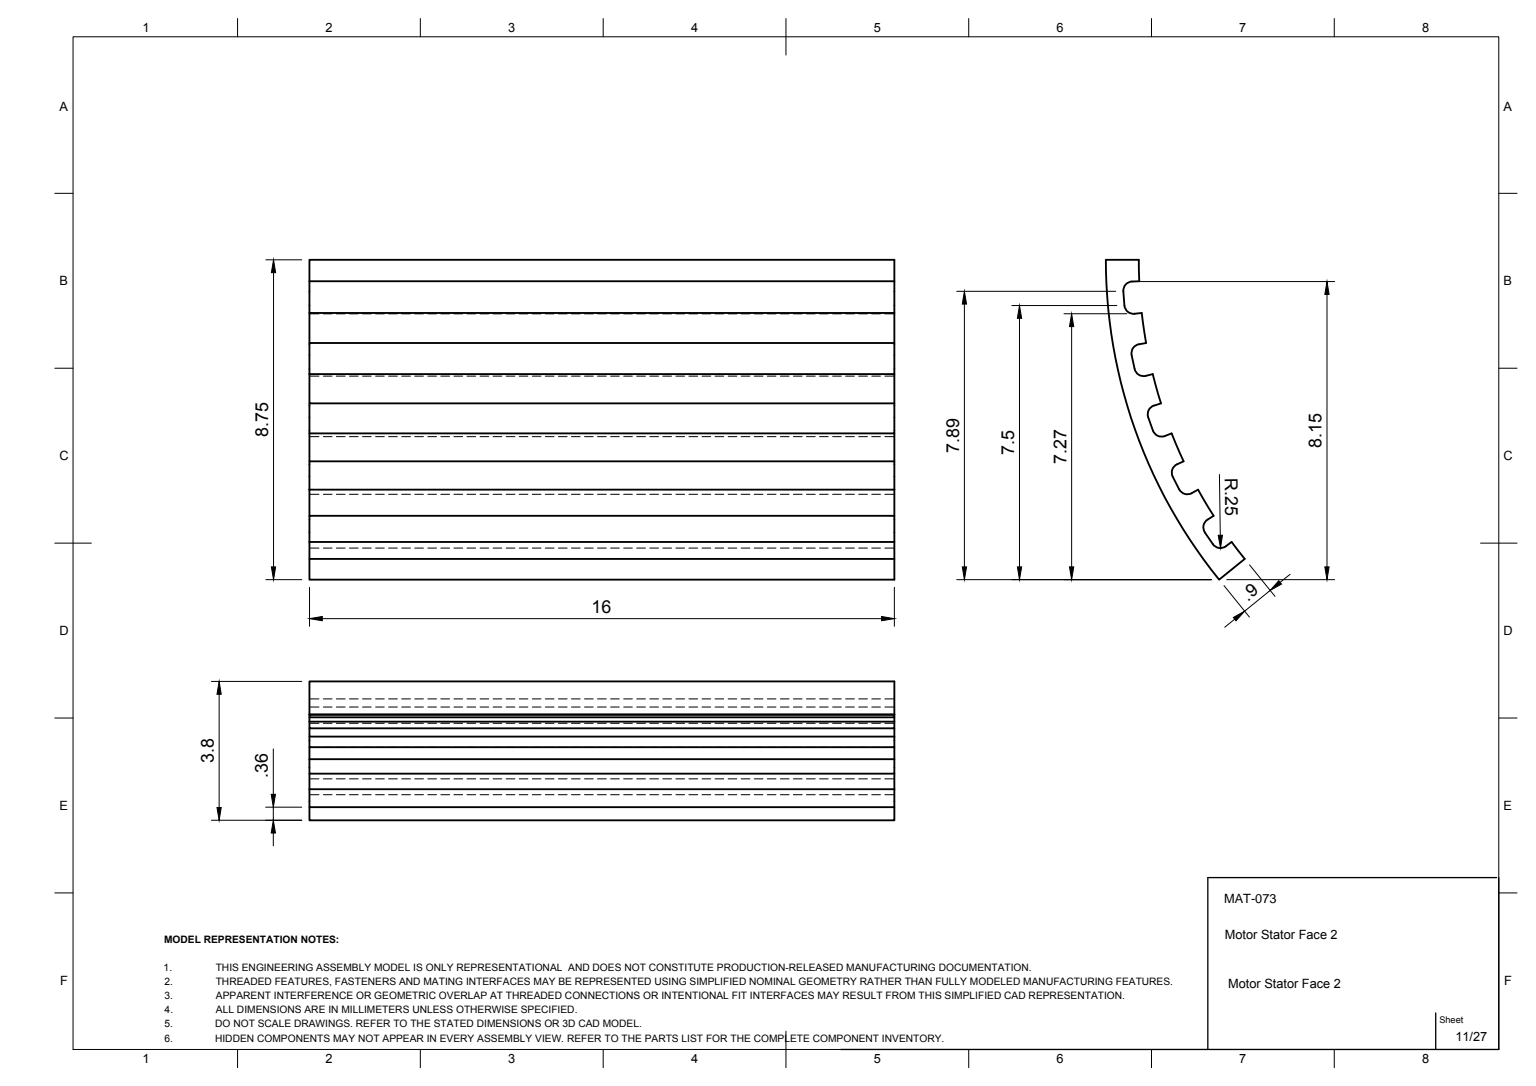
ISO-10303-21;
HEADER;
/* Generated by software containing ST-Developer
 * from STEP Tools, Inc. (www.steptools.com) 
 */

FILE_DESCRIPTION(
/* description */ ('CAx-IF Rec.Pracs.---Representation and Presentation of Product Manufa
cturing Information (PMI)---4.0---2014-10-13'),
/* implementation_level */ '2;1');

FILE_NAME(
/* name */ 'Motor Stator Face 2.step',
/* time_stamp */ '2026-10-24T18:52:33-07:00',
/* author */ (''),
/* organization */ (''),
/* preprocessor_version */ 'ST-DEVELOPER v20.2',
/* originating_system */ 'Autodesk Translation Framework v15.17.0.0',
/* authorisation */ '');

FILE_SCHEMA (('AP242_MANAGED_MODEL_BASED_3D_ENGINEERING_MIM_LF { 1 0 10303 442 2 1 4 }'));
ENDSEC;

DATA;
#10=MECHANICAL_DESIGN_GEOMETRIC_PRESENTATION_REPRESENTATION('',(#424),#34876);
#358=SHAPE_REPRESENTATION_RELATIONSHIP('SRR','None',#34995,#391);
#391=ADVANCED_BREP_SHAPE_REPRESENTATION('',(#457),#34853);
#424=STYLED_ITEM('',(#35166),#457);
#457=MANIFOLD_SOLID_BREP('Motor Stator Face 2',#19564);
#802=PLANE('',#20894);
#803=PLANE('',#20904);
#804=PLANE('',#20914);
#805=PLANE('',#20924);
#806=PLANE('',#20934);
#807=PLANE('',#20935);
#808=PLANE('',#20936);
#809=PLANE('',#20937);
#810=PLANE('',#20938);
#811=PLANE('',#20945);
#812=PLANE('',#20955);
#813=PLANE('',#20958);
#814=PLANE('',#20961);
#815=PLANE('',#20964);
#1709=LINE('',#31107,#3308);
#1710=LINE('',#31110,#3309);
#1711=LINE('',#31115,#3310);
#1712=LINE('',#31121,#3311);
#1713=LINE('',#31125,#3312);
#1714=LINE('',#31127,#3313);
#1715=LINE('',#31128,#3314);
#1716=LINE('',#31134,#3315);
#1717=LINE('',#31137,#3316);
#1718=LINE('',#31142,#3317);
#1719=LINE('',#31148,#3318);
#1720=LINE('',#31152,#3319);
#1721=LINE('',#31154,#3320);
#1722=LINE('',#31155,#3321);
#1723=LINE('',#31161,#3322);
#1724=LINE('',#31164,#3323);
#1725=LINE('',#31169,#3324);
#1726=LINE('',#31175,#3325);
#1727=LINE('',#31179,#3326);
#1728=LINE('',#31181,#3327);
#1729=LINE('',#31182,#3328);
#1730=LINE('',#31188,#3329);
#1731=LINE('',#31191,#3330);
#1732=LINE('',#31196,#3331);
#1733=LINE('',#31202,#3332);
#1734=LINE('',#31206,#3333);
#1735=LINE('',#31208,#3334);
#1736=LINE('',#31209,#3335);
#1737=LINE('',#31215,#3336);
#1738=LINE('',#31218,#3337);
#1739=LINE('',#31223,#3338);
#1740=LINE('',#31229,#3339);
#1741=LINE('',#31233,#3340);
#1742=LINE('',#31235,#3341);
#1743=LINE('',#31236,#3342);
#1744=LINE('',#31239,#3343);
#1745=LINE('',#31241,#3344);
#1746=LINE('',#31242,#3345);
#1747=LINE('',#31245,#3346);
#1748=LINE('',#31247,#3347);
#1749=LINE('',#31248,#3348);
#1750=LINE('',#31251,#3349);
#1751=LINE('',#31253,#3350);
#1752=LINE('',#31254,#3351);
#1753=LINE('',#31257,#3352);
#1754=LINE('',#31259,#3353);
#1755=LINE('',#31260,#3354);
#1756=LINE('',#31265,#3355);
#1757=LINE('',#31272,#3356);
#1758=LINE('',#31276,#3357);
#1759=LINE('',#31281,#3358);
#1760=LINE('',#31286,#3359);
#1761=LINE('',#31289,#3360);
#1762=LINE('',#31292,#3361);
#1763=LINE('',#31297,#3362);
#1764=LINE('',#31298,#3363);
#1765=LINE('',#31302,#3364);
#1766=LINE('',#31304,#3365);
#3308=VECTOR('',#24756,1.);
#3309=VECTOR('',#24759,1.);
#3310=VECTOR('',#24764,1.);
#3311=VECTOR('',#24771,1.);
#3312=VECTOR('',#24776,1.);
#3313=VECTOR('',#24777,1.);
#3314=VECTOR('',#24778,1.);
#3315=VECTOR('',#24783,1.);
#3316=VECTOR('',#24786,1.);
#3317=VECTOR('',#24791,1.);
#3318=VECTOR('',#24798,1.);
#3319=VECTOR('',#24803,1.);
#3320=VECTOR('',#24804,1.);
#3321=VECTOR('',#24805,1.);
#3322=VECTOR('',#24810,1.);
#3323=VECTOR('',#24813,1.);
#3324=VECTOR('',#24818,1.);
#3325=VECTOR('',#24825,1.);
#3326=VECTOR('',#24830,1.);
#3327=VECTOR('',#24831,1.);
#3328=VECTOR('',#24832,1.);
#3329=VECTOR('',#24837,1.);
#3330=VECTOR('',#24840,1.);
#3331=VECTOR('',#24845,1.);
#3332=VECTOR('',#24852,1.);
#3333=VECTOR('',#24857,1.);
#3334=VECTOR('',#24858,1.);
#3335=VECTOR('',#24859,1.);
#3336=VECTOR('',#24864,1.);
#3337=VECTOR('',#24867,1.);
#3338=VECTOR('',#24872,1.);
#3339=VECTOR('',#24879,1.);
#3340=VECTOR('',#24884,1.);
#3341=VECTOR('',#24885,1.);
#3342=VECTOR('',#24886,1.);
#3343=VECTOR('',#24889,1.);
#3344=VECTOR('',#24890,1.);
#3345=VECTOR('',#24891,1.);
#3346=VECTOR('',#24894,1.);
#3347=VECTOR('',#24895,1.);
#3348=VECTOR('',#24896,1.);
#3349=VECTOR('',#24899,1.);
#3350=VECTOR('',#24900,1.);
#3351=VECTOR('',#24901,1.);
#3352=VECTOR('',#24904,1.);
#3353=VECTOR('',#24905,1.);
#3354=VECTOR('',#24906,1.);
#3355=VECTOR('',#24911,1.);
#3356=VECTOR('',#24922,1.);
#3357=VECTOR('',#24925,1.);
#3358=VECTOR('',#24932,1.);
#3359=VECTOR('',#24939,1.);
#3360=VECTOR('',#24942,1.);
#3361=VECTOR('',#24947,1.);
#3362=VECTOR('',#24954,1.);
#3363=VECTOR('',#24955,1.);
#3364=VECTOR('',#24960,1.);
#3365=VECTOR('',#24963,1.);
#4482=CYLINDRICAL_SURFACE('',#20885,0.00025);
#4483=CYLINDRICAL_SURFACE('',#20888,0.01345);
#4484=CYLINDRICAL_SURFACE('',#20891,0.00025);
#4485=CYLINDRICAL_SURFACE('',#20895,0.00025);
#4486=CYLINDRICAL_SURFACE('',#20898,0.01345);
#4487=CYLINDRICAL_SURFACE('',#20901,0.00025);
#4488=CYLINDRICAL_SURFACE('',#20905,0.00025);
#4489=CYLINDRICAL_SURFACE('',#20908,0.01345);
#4490=CYLINDRICAL_SURFACE('',#20911,0.00025);
#4491=CYLINDRICAL_SURFACE('',#20915,0.00025);
#4492=CYLINDRICAL_SURFACE('',#20918,0.01345);
#4493=CYLINDRICAL_SURFACE('',#20921,0.00025);
#4494=CYLINDRICAL_SURFACE('',#20925,0.00025);
#4495=CYLINDRICAL_SURFACE('',#20928,0.01345);
#4496=CYLINDRICAL_SURFACE('',#20931,0.00025);
#4497=CYLINDRICAL_SURFACE('',#20939,0.013);
#4498=CYLINDRICAL_SURFACE('',#20942,0.013);
#4499=CYLINDRICAL_SURFACE('',#20951,0.013);
#4500=CYLINDRICAL_SURFACE('',#20953,0.013);
#4501=CYLINDRICAL_SURFACE('',#20956,0.013);
#4502=CYLINDRICAL_SURFACE('',#20959,0.0139);
#4503=CYLINDRICAL_SURFACE('',#20962,0.013);
#5216=FACE_OUTER_BOUND('',#6300,.T.);
#5217=FACE_OUTER_BOUND('',#6301,.T.);
#5218=FACE_OUTER_BOUND('',#6302,.T.);
#5219=FACE_OUTER_BOUND('',#6303,.T.);
#5220=FACE_OUTER_BOUND('',#6304,.T.);
#5221=FACE_OUTER_BOUND('',#6305,.T.);
#5222=FACE_OUTER_BOUND('',#6306,.T.);
#5223=FACE_OUTER_BOUND('',#6307,.T.);
#5224=FACE_OUTER_BOUND('',#6308,.T.);
#5225=FACE_OUTER_BOUND('',#6309,.T.);
#5226=FACE_OUTER_BOUND('',#6310,.T.);
#5227=FACE_OUTER_BOUND('',#6311,.T.);
#5228=FACE_OUTER_BOUND('',#6312,.T.);
#5229=FACE_OUTER_BOUND('',#6313,.T.);
#5230=FACE_OUTER_BOUND('',#6314,.T.);
#5231=FACE_OUTER_BOUND('',#6315,.T.);
#5232=FACE_OUTER_BOUND('',#6316,.T.);
#5233=FACE_OUTER_BOUND('',#6317,.T.);
#5234=FACE_OUTER_BOUND('',#6318,.T.);
#5235=FACE_OUTER_BOUND('',#6319,.T.);
#5236=FACE_OUTER_BOUND('',#6320,.T.);
#5237=FACE_OUTER_BOUND('',#6321,.T.);
#5238=FACE_OUTER_BOUND('',#6322,.T.);
#5239=FACE_OUTER_BOUND('',#6323,.T.);
#5240=FACE_OUTER_BOUND('',#6324,.T.);
#5241=FACE_OUTER_BOUND('',#6325,.T.);
#5242=FACE_OUTER_BOUND('',#6326,.T.);
#5243=FACE_OUTER_BOUND('',#6327,.T.);
#5244=FACE_OUTER_BOUND('',#6328,.T.);
#5245=FACE_OUTER_BOUND('',#6329,.T.);
#5246=FACE_OUTER_BOUND('',#6330,.T.);
#5247=FACE_OUTER_BOUND('',#6331,.T.);
#5248=FACE_OUTER_BOUND('',#6332,.T.);
#5249=FACE_OUTER_BOUND('',#6333,.T.);
#5250=FACE_OUTER_BOUND('',#6334,.T.);
#5251=FACE_OUTER_BOUND('',#6335,.T.);
#6300=EDGE_LOOP('',(#15096,#15097,#15098,#15099));
#6301=EDGE_LOOP('',(#15100,#15101,#15102,#15103));
#6302=EDGE_LOOP('',(#15104,#15105,#15106,#15107));
#6303=EDGE_LOOP('',(#15108,#15109,#15110,#15111));
#6304=EDGE_LOOP('',(#15112,#15113,#15114,#15115));
#6305=EDGE_LOOP('',(#15116,#15117,#15118,#15119));
#6306=EDGE_LOOP('',(#15120,#15121,#15122,#15123));
#6307=EDGE_LOOP('',(#15124,#15125,#15126,#15127));
#6308=EDGE_LOOP('',(#15128,#15129,#15130,#15131));
#6309=EDGE_LOOP('',(#15132,#15133,#15134,#15135));
#6310=EDGE_LOOP('',(#15136,#15137,#15138,#15139));
#6311=EDGE_LOOP('',(#15140,#15141,#15142,#15143));
#6312=EDGE_LOOP('',(#15144,#15145,#15146,#15147));
#6313=EDGE_LOOP('',(#15148,#15149,#15150,#15151));
#6314=EDGE_LOOP('',(#15152,#15153,#15154,#15155));
#6315=EDGE_LOOP('',(#15156,#15157,#15158,#15159));
#6316=EDGE_LOOP('',(#15160,#15161,#15162,#15163));
#6317=EDGE_LOOP('',(#15164,#15165,#15166,#15167));
#6318=EDGE_LOOP('',(#15168,#15169,#15170,#15171));
#6319=EDGE_LOOP('',(#15172,#15173,#15174,#15175));
#6320=EDGE_LOOP('',(#15176,#15177,#15178,#15179));
#6321=EDGE_LOOP('',(#15180,#15181,#15182,#15183));
#6322=EDGE_LOOP('',(#15184,#15185,#15186,#15187));
#6323=EDGE_LOOP('',(#15188,#15189,#15190,#15191));
#6324=EDGE_LOOP('',(#15192,#15193,#15194,#15195));
#6325=EDGE_LOOP('',(#15196,#15197,#15198,#15199));
#6326=EDGE_LOOP('',(#15200,#15201,#15202,#15203,#15204,#15205,#15206,#15207,
#15208,#15209,#15210,#15211,#15212,#15213,#15214,#15215,#15216,#15217,#15218,
#15219,#15220,#15221,#15222,#15223,#15224,#15225,#15226,#15227,#15228,#15229,
#15230,#15231,#15232,#15233));
#6327=EDGE_LOOP('',(#15234,#15235,#15236,#15237));
#6328=EDGE_LOOP('',(#15238,#15239,#15240,#15241));
#6329=EDGE_LOOP('',(#15242,#15243,#15244,#15245));
#6330=EDGE_LOOP('',(#15246,#15247,#15248,#15249));
#6331=EDGE_LOOP('',(#15250,#15251,#15252,#15253));
#6332=EDGE_LOOP('',(#15254,#15255,#15256,#15257));
#6333=EDGE_LOOP('',(#15258,#15259,#15260,#15261));
#6334=EDGE_LOOP('',(#15262,#15263,#15264,#15265));
#6335=EDGE_LOOP('',(#15266,#15267,#15268,#15269,#15270,#15271,#15272,#15273,
#15274,#15275,#15276,#15277,#15278,#15279,#15280,#15281,#15282,#15283,#15284,
#15285,#15286,#15287,#15288,#15289,#15290,#15291,#15292,#15293,#15294,#15295,
#15296,#15297,#15298,#15299));
#7404=CIRCLE('',#20886,0.000250000000013569);
#7405=CIRCLE('',#20887,0.000250000000013569);
#7406=CIRCLE('',#20889,0.0134500000000125);
#7407=CIRCLE('',#20890,0.0134500000000125);
#7408=CIRCLE('',#20892,0.000250000000013744);
#7409=CIRCLE('',#20893,0.000250000000013744);
#7410=CIRCLE('',#20896,0.000250000000013973);
#7411=CIRCLE('',#20897,0.000250000000013973);
#7412=CIRCLE('',#20899,0.0134500000000115);
#7413=CIRCLE('',#20900,0.0134500000000115);
#7414=CIRCLE('',#20902,0.000250000000014062);
#7415=CIRCLE('',#20903,0.000250000000014062);
#7416=CIRCLE('',#20906,0.000250000000014138);
#7417=CIRCLE('',#20907,0.000250000000014138);
#7418=CIRCLE('',#20909,0.0134500000000103);
#7419=CIRCLE('',#20910,0.0134500000000103);
#7420=CIRCLE('',#20912,0.000250000000014138);
#7421=CIRCLE('',#20913,0.000250000000014138);
#7422=CIRCLE('',#20916,0.000250000000014062);
#7423=CIRCLE('',#20917,0.000250000000014062);
#7424=CIRCLE('',#20919,0.0134500000000109);
#7425=CIRCLE('',#20920,0.0134500000000109);
#7426=CIRCLE('',#20922,0.000250000000013973);
#7427=CIRCLE('',#20923,0.000250000000013973);
#7428=CIRCLE('',#20926,0.000250000000013744);
#7429=CIRCLE('',#20927,0.000250000000013744);
#7430=CIRCLE('',#20929,0.013450000000012);
#7431=CIRCLE('',#20930,0.013450000000012);
#7432=CIRCLE('',#20932,0.000250000000013569);
#7433=CIRCLE('',#20933,0.000250000000013569);
#7434=CIRCLE('',#20940,0.0130000000000128);
#7435=CIRCLE('',#20941,0.0130000000000128);
#7436=CIRCLE('',#20943,0.0130000000000128);
#7437=CIRCLE('',#20944,0.0130000000000128);
#7438=CIRCLE('',#20946,0.0139000000000128);
#7439=CIRCLE('',#20947,0.0130000000000128);
#7440=CIRCLE('',#20948,0.0130000000000128);
#7441=CIRCLE('',#20949,0.0130000000000128);
#7442=CIRCLE('',#20950,0.0130000000000128);
#7443=CIRCLE('',#20952,0.0130000000000128);
#7444=CIRCLE('',#20954,0.0130000000000128);
#7445=CIRCLE('',#20957,0.0130000000000128);
#7446=CIRCLE('',#20960,0.0139000000000128);
#7447=CIRCLE('',#20963,0.0130000000000128);
#8832=VERTEX_POINT('',#31103);
#8833=VERTEX_POINT('',#31104);
#8834=VERTEX_POINT('',#31106);
#8835=VERTEX_POINT('',#31108);
#8836=VERTEX_POINT('',#31112);
#8837=VERTEX_POINT('',#31114);
#8838=VERTEX_POINT('',#31118);
#8839=VERTEX_POINT('',#31120);
#8840=VERTEX_POINT('',#31124);
#8841=VERTEX_POINT('',#31126);
#8842=VERTEX_POINT('',#31130);
#8843=VERTEX_POINT('',#31131);
#8844=VERTEX_POINT('',#31133);
#8845=VERTEX_POINT('',#31135);
#8846=VERTEX_POINT('',#31139);
#8847=VERTEX_POINT('',#31141);
#8848=VERTEX_POINT('',#31145);
#8849=VERTEX_POINT('',#31147);
#8850=VERTEX_POINT('',#31151);
#8851=VERTEX_POINT('',#31153);
#8852=VERTEX_POINT('',#31157);
#8853=VERTEX_POINT('',#31158);
#8854=VERTEX_POINT('',#31160);
#8855=VERTEX_POINT('',#31162);
#8856=VERTEX_POINT('',#31166);
#8857=VERTEX_POINT('',#31168);
#8858=VERTEX_POINT('',#31172);
#8859=VERTEX_POINT('',#31174);
#8860=VERTEX_POINT('',#31178);
#8861=VERTEX_POINT('',#31180);
#8862=VERTEX_POINT('',#31184);
#8863=VERTEX_POINT('',#31185);
#8864=VERTEX_POINT('',#31187);
#8865=VERTEX_POINT('',#31189);
#8866=VERTEX_POINT('',#31193);
#8867=VERTEX_POINT('',#31195);
#8868=VERTEX_POINT('',#31199);
#8869=VERTEX_POINT('',#31201);
#8870=VERTEX_POINT('',#31205);
#8871=VERTEX_POINT('',#31207);
#8872=VERTEX_POINT('',#31211);
#8873=VERTEX_POINT('',#31212);
#8874=VERTEX_POINT('',#31214);
#8875=VERTEX_POINT('',#31216);
#8876=VERTEX_POINT('',#31220);
#8877=VERTEX_POINT('',#31222);
#8878=VERTEX_POINT('',#31226);
#8879=VERTEX_POINT('',#31228);
#8880=VERTEX_POINT('',#31232);
#8881=VERTEX_POINT('',#31234);
#8882=VERTEX_POINT('',#31238);
#8883=VERTEX_POINT('',#31240);
#8884=VERTEX_POINT('',#31244);
#8885=VERTEX_POINT('',#31246);
#8886=VERTEX_POINT('',#31250);
#8887=VERTEX_POINT('',#31252);
#8888=VERTEX_POINT('',#31256);
#8889=VERTEX_POINT('',#31258);
#8890=VERTEX_POINT('',#31262);
#8891=VERTEX_POINT('',#31264);
#8892=VERTEX_POINT('',#31271);
#8893=VERTEX_POINT('',#31273);
#8894=VERTEX_POINT('',#31275);
#8895=VERTEX_POINT('',#31279);
#8896=VERTEX_POINT('',#31284);
#8897=VERTEX_POINT('',#31288);
#8898=VERTEX_POINT('',#31296);
#8899=VERTEX_POINT('',#31300);
#11106=EDGE_CURVE('',#8832,#8833,#7404,.T.);
#11107=EDGE_CURVE('',#8833,#8834,#1709,.T.);
#11108=EDGE_CURVE('',#8834,#8835,#7405,.T.);
#11109=EDGE_CURVE('',#8835,#8832,#1710,.T.);
#11110=EDGE_CURVE('',#8836,#8833,#7406,.T.);
#11111=EDGE_CURVE('',#8837,#8836,#1711,.T.);
#11112=EDGE_CURVE('',#8834,#8837,#7407,.T.);
#11113=EDGE_CURVE('',#8836,#8838,#7408,.T.);
#11114=EDGE_CURVE('',#8838,#8839,#1712,.T.);
#11115=EDGE_CURVE('',#8839,#8837,#7409,.T.);
#11116=EDGE_CURVE('',#8840,#8838,#1713,.T.);
#11117=EDGE_CURVE('',#8841,#8840,#1714,.T.);
#11118=EDGE_CURVE('',#8839,#8841,#1715,.T.);
#11119=EDGE_CURVE('',#8842,#8843,#7410,.T.);
#11120=EDGE_CURVE('',#8843,#8844,#1716,.T.);
#11121=EDGE_CURVE('',#8844,#8845,#7411,.T.);
#11122=EDGE_CURVE('',#8845,#8842,#1717,.T.);
#11123=EDGE_CURVE('',#8846,#8843,#7412,.T.);
#11124=EDGE_CURVE('',#8847,#8846,#1718,.T.);
#11125=EDGE_CURVE('',#8844,#8847,#7413,.T.);
#11126=EDGE_CURVE('',#8846,#8848,#7414,.T.);
#11127=EDGE_CURVE('',#8848,#8849,#1719,.T.);
#11128=EDGE_CURVE('',#8849,#8847,#7415,.T.);
#11129=EDGE_CURVE('',#8850,#8848,#1720,.T.);
#11130=EDGE_CURVE('',#8851,#8850,#1721,.T.);
#11131=EDGE_CURVE('',#8849,#8851,#1722,.T.);
#11132=EDGE_CURVE('',#8852,#8853,#7416,.T.);
#11133=EDGE_CURVE('',#8853,#8854,#1723,.T.);
#11134=EDGE_CURVE('',#8854,#8855,#7417,.T.);
#11135=EDGE_CURVE('',#8855,#8852,#1724,.T.);
#11136=EDGE_CURVE('',#8856,#8853,#7418,.T.);
#11137=EDGE_CURVE('',#8857,#8856,#1725,.T.);
#11138=EDGE_CURVE('',#8854,#8857,#7419,.T.);
#11139=EDGE_CURVE('',#8856,#8858,#7420,.T.);
#11140=EDGE_CURVE('',#8858,#8859,#1726,.T.);
#11141=EDGE_CURVE('',#8859,#8857,#7421,.T.);
#11142=EDGE_CURVE('',#8860,#8858,#1727,.T.);
#11143=EDGE_CURVE('',#8861,#8860,#1728,.T.);
#11144=EDGE_CURVE('',#8859,#8861,#1729,.T.);
#11145=EDGE_CURVE('',#8862,#8863,#7422,.T.);
#11146=EDGE_CURVE('',#8863,#8864,#1730,.T.);
#11147=EDGE_CURVE('',#8864,#8865,#7423,.T.);
#11148=EDGE_CURVE('',#8865,#8862,#1731,.T.);
#11149=EDGE_CURVE('',#8866,#8863,#7424,.T.);
#11150=EDGE_CURVE('',#8867,#8866,#1732,.T.);
#11151=EDGE_CURVE('',#8864,#8867,#7425,.T.);
#11152=EDGE_CURVE('',#8866,#8868,#7426,.T.);
#11153=EDGE_CURVE('',#8868,#8869,#1733,.T.);
#11154=EDGE_CURVE('',#8869,#8867,#7427,.T.);
#11155=EDGE_CURVE('',#8870,#8868,#1734,.T.);
#11156=EDGE_CURVE('',#8871,#8870,#1735,.T.);
#11157=EDGE_CURVE('',#8869,#8871,#1736,.T.);
#11158=EDGE_CURVE('',#8872,#8873,#7428,.T.);
#11159=EDGE_CURVE('',#8873,#8874,#1737,.T.);
#11160=EDGE_CURVE('',#8874,#8875,#7429,.T.);
#11161=EDGE_CURVE('',#8875,#8872,#1738,.T.);
#11162=EDGE_CURVE('',#8876,#8873,#7430,.T.);
#11163=EDGE_CURVE('',#8877,#8876,#1739,.T.);
#11164=EDGE_CURVE('',#8874,#8877,#7431,.T.);
#11165=EDGE_CURVE('',#8876,#8878,#7432,.T.);
#11166=EDGE_CURVE('',#8878,#8879,#1740,.T.);
#11167=EDGE_CURVE('',#8879,#8877,#7433,.T.);
#11168=EDGE_CURVE('',#8880,#8878,#1741,.T.);
#11169=EDGE_CURVE('',#8881,#8880,#1742,.T.);
#11170=EDGE_CURVE('',#8879,#8881,#1743,.T.);
#11171=EDGE_CURVE('',#8882,#8875,#1744,.T.);
#11172=EDGE_CURVE('',#8883,#8882,#1745,.T.);
#11173=EDGE_CURVE('',#8872,#8883,#1746,.T.);
#11174=EDGE_CURVE('',#8884,#8865,#1747,.T.);
#11175=EDGE_CURVE('',#8885,#8884,#1748,.T.);
#11176=EDGE_CURVE('',#8862,#8885,#1749,.T.);
#11177=EDGE_CURVE('',#8886,#8845,#1750,.T.);
#11178=EDGE_CURVE('',#8887,#8886,#1751,.T.);
#11179=EDGE_CURVE('',#8842,#8887,#1752,.T.);
#11180=EDGE_CURVE('',#8888,#8835,#1753,.T.);
#11181=EDGE_CURVE('',#8889,#8888,#1754,.T.);
#11182=EDGE_CURVE('',#8832,#8889,#1755,.T.);
#11183=EDGE_CURVE('',#8890,#8880,#7434,.T.);
#11184=EDGE_CURVE('',#8890,#8891,#1756,.T.);
#11185=EDGE_CURVE('',#8881,#8891,#7435,.T.);
#11186=EDGE_CURVE('',#8861,#8884,#7436,.T.);
#11187=EDGE_CURVE('',#8885,#8860,#7437,.T.);
#11188=EDGE_CURVE('',#8891,#8892,#1757,.T.);
#11189=EDGE_CURVE('',#8892,#8893,#7438,.T.);
#11190=EDGE_CURVE('',#8893,#8894,#1758,.T.);
#11191=EDGE_CURVE('',#8894,#8888,#7439,.T.);
#11192=EDGE_CURVE('',#8841,#8886,#7440,.T.);
#11193=EDGE_CURVE('',#8851,#8895,#7441,.T.);
#11194=EDGE_CURVE('',#8895,#8855,#1759,.T.);
#11195=EDGE_CURVE('',#8871,#8882,#7442,.T.);
#11196=EDGE_CURVE('',#8896,#8850,#7443,.T.);
#11197=EDGE_CURVE('',#8896,#8895,#1760,.T.);
#11198=EDGE_CURVE('',#8894,#8897,#1761,.T.);
#11199=EDGE_CURVE('',#8889,#8897,#7444,.T.);
#11200=EDGE_CURVE('',#8852,#8896,#1762,.T.);
#11201=EDGE_CURVE('',#8883,#8870,#7445,.T.);
#11202=EDGE_CURVE('',#8898,#8890,#1763,.T.);
#11203=EDGE_CURVE('',#8892,#8898,#1764,.T.);
#11204=EDGE_CURVE('',#8899,#8898,#7446,.T.);
#11205=EDGE_CURVE('',#8893,#8899,#1765,.T.);
#11206=EDGE_CURVE('',#8897,#8899,#1766,.T.);
#11207=EDGE_CURVE('',#8887,#8840,#7447,.T.);
#15096=ORIENTED_EDGE('',*,*,#11106,.T.);
#15097=ORIENTED_EDGE('',*,*,#11107,.T.);
#15098=ORIENTED_EDGE('',*,*,#11108,.T.);
#15099=ORIENTED_EDGE('',*,*,#11109,.T.);
#15100=ORIENTED_EDGE('',*,*,#11107,.F.);
#15101=ORIENTED_EDGE('',*,*,#11110,.F.);
#15102=ORIENTED_EDGE('',*,*,#11111,.F.);
#15103=ORIENTED_EDGE('',*,*,#11112,.F.);
#15104=ORIENTED_EDGE('',*,*,#11113,.T.);
#15105=ORIENTED_EDGE('',*,*,#11114,.T.);
#15106=ORIENTED_EDGE('',*,*,#11115,.T.);
#15107=ORIENTED_EDGE('',*,*,#11111,.T.);
#15108=ORIENTED_EDGE('',*,*,#11114,.F.);
#15109=ORIENTED_EDGE('',*,*,#11116,.F.);
#15110=ORIENTED_EDGE('',*,*,#11117,.F.);
#15111=ORIENTED_EDGE('',*,*,#11118,.F.);
#15112=ORIENTED_EDGE('',*,*,#11119,.T.);
#15113=ORIENTED_EDGE('',*,*,#11120,.T.);
#15114=ORIENTED_EDGE('',*,*,#11121,.T.);
#15115=ORIENTED_EDGE('',*,*,#11122,.T.);
#15116=ORIENTED_EDGE('',*,*,#11120,.F.);
#15117=ORIENTED_EDGE('',*,*,#11123,.F.);
#15118=ORIENTED_EDGE('',*,*,#11124,.F.);
#15119=ORIENTED_EDGE('',*,*,#11125,.F.);
#15120=ORIENTED_EDGE('',*,*,#11126,.T.);
#15121=ORIENTED_EDGE('',*,*,#11127,.T.);
#15122=ORIENTED_EDGE('',*,*,#11128,.T.);
#15123=ORIENTED_EDGE('',*,*,#11124,.T.);
#15124=ORIENTED_EDGE('',*,*,#11127,.F.);
#15125=ORIENTED_EDGE('',*,*,#11129,.F.);
#15126=ORIENTED_EDGE('',*,*,#11130,.F.);
#15127=ORIENTED_EDGE('',*,*,#11131,.F.);
#15128=ORIENTED_EDGE('',*,*,#11132,.T.);
#15129=ORIENTED_EDGE('',*,*,#11133,.T.);
#15130=ORIENTED_EDGE('',*,*,#11134,.T.);
#15131=ORIENTED_EDGE('',*,*,#11135,.T.);
#15132=ORIENTED_EDGE('',*,*,#11133,.F.);
#15133=ORIENTED_EDGE('',*,*,#11136,.F.);
#15134=ORIENTED_EDGE('',*,*,#11137,.F.);
#15135=ORIENTED_EDGE('',*,*,#11138,.F.);
#15136=ORIENTED_EDGE('',*,*,#11139,.T.);
#15137=ORIENTED_EDGE('',*,*,#11140,.T.);
#15138=ORIENTED_EDGE('',*,*,#11141,.T.);
#15139=ORIENTED_EDGE('',*,*,#11137,.T.);
#15140=ORIENTED_EDGE('',*,*,#11140,.F.);
#15141=ORIENTED_EDGE('',*,*,#11142,.F.);
#15142=ORIENTED_EDGE('',*,*,#11143,.F.);
#15143=ORIENTED_EDGE('',*,*,#11144,.F.);
#15144=ORIENTED_EDGE('',*,*,#11145,.T.);
#15145=ORIENTED_EDGE('',*,*,#11146,.T.);
#15146=ORIENTED_EDGE('',*,*,#11147,.T.);
#15147=ORIENTED_EDGE('',*,*,#11148,.T.);
#15148=ORIENTED_EDGE('',*,*,#11146,.F.);
#15149=ORIENTED_EDGE('',*,*,#11149,.F.);
#15150=ORIENTED_EDGE('',*,*,#11150,.F.);
#15151=ORIENTED_EDGE('',*,*,#11151,.F.);
#15152=ORIENTED_EDGE('',*,*,#11152,.T.);
#15153=ORIENTED_EDGE('',*,*,#11153,.T.);
#15154=ORIENTED_EDGE('',*,*,#11154,.T.);
#15155=ORIENTED_EDGE('',*,*,#11150,.T.);
#15156=ORIENTED_EDGE('',*,*,#11153,.F.);
#15157=ORIENTED_EDGE('',*,*,#11155,.F.);
#15158=ORIENTED_EDGE('',*,*,#11156,.F.);
#15159=ORIENTED_EDGE('',*,*,#11157,.F.);
#15160=ORIENTED_EDGE('',*,*,#11158,.T.);
#15161=ORIENTED_EDGE('',*,*,#11159,.T.);
#15162=ORIENTED_EDGE('',*,*,#11160,.T.);
#15163=ORIENTED_EDGE('',*,*,#11161,.T.);
#15164=ORIENTED_EDGE('',*,*,#11159,.F.);
#15165=ORIENTED_EDGE('',*,*,#11162,.F.);
#15166=ORIENTED_EDGE('',*,*,#11163,.F.);
#15167=ORIENTED_EDGE('',*,*,#11164,.F.);
#15168=ORIENTED_EDGE('',*,*,#11165,.T.);
#15169=ORIENTED_EDGE('',*,*,#11166,.T.);
#15170=ORIENTED_EDGE('',*,*,#11167,.T.);
#15171=ORIENTED_EDGE('',*,*,#11163,.T.);
#15172=ORIENTED_EDGE('',*,*,#11166,.F.);
#15173=ORIENTED_EDGE('',*,*,#11168,.F.);
#15174=ORIENTED_EDGE('',*,*,#11169,.F.);
#15175=ORIENTED_EDGE('',*,*,#11170,.F.);
#15176=ORIENTED_EDGE('',*,*,#11161,.F.);
#15177=ORIENTED_EDGE('',*,*,#11171,.F.);
#15178=ORIENTED_EDGE('',*,*,#11172,.F.);
#15179=ORIENTED_EDGE('',*,*,#11173,.F.);
#15180=ORIENTED_EDGE('',*,*,#11148,.F.);
#15181=ORIENTED_EDGE('',*,*,#11174,.F.);
#15182=ORIENTED_EDGE('',*,*,#11175,.F.);
#15183=ORIENTED_EDGE('',*,*,#11176,.F.);
#15184=ORIENTED_EDGE('',*,*,#11122,.F.);
#15185=ORIENTED_EDGE('',*,*,#11177,.F.);
#15186=ORIENTED_EDGE('',*,*,#11178,.F.);
#15187=ORIENTED_EDGE('',*,*,#11179,.F.);
#15188=ORIENTED_EDGE('',*,*,#11109,.F.);
#15189=ORIENTED_EDGE('',*,*,#11180,.F.);
#15190=ORIENTED_EDGE('',*,*,#11181,.F.);
#15191=ORIENTED_EDGE('',*,*,#11182,.F.);
#15192=ORIENTED_EDGE('',*,*,#11169,.T.);
#15193=ORIENTED_EDGE('',*,*,#11183,.F.);
#15194=ORIENTED_EDGE('',*,*,#11184,.T.);
#15195=ORIENTED_EDGE('',*,*,#11185,.F.);
#15196=ORIENTED_EDGE('',*,*,#11175,.T.);
#15197=ORIENTED_EDGE('',*,*,#11186,.F.);
#15198=ORIENTED_EDGE('',*,*,#11143,.T.);
#15199=ORIENTED_EDGE('',*,*,#11187,.F.);
#15200=ORIENTED_EDGE('',*,*,#11171,.T.);
#15201=ORIENTED_EDGE('',*,*,#11160,.F.);
#15202=ORIENTED_EDGE('',*,*,#11164,.T.);
#15203=ORIENTED_EDGE('',*,*,#11167,.F.);
#15204=ORIENTED_EDGE('',*,*,#11170,.T.);
#15205=ORIENTED_EDGE('',*,*,#11185,.T.);
#15206=ORIENTED_EDGE('',*,*,#11188,.T.);
#15207=ORIENTED_EDGE('',*,*,#11189,.T.);
#15208=ORIENTED_EDGE('',*,*,#11190,.T.);
#15209=ORIENTED_EDGE('',*,*,#11191,.T.);
#15210=ORIENTED_EDGE('',*,*,#11180,.T.);
#15211=ORIENTED_EDGE('',*,*,#11108,.F.);
#15212=ORIENTED_EDGE('',*,*,#11112,.T.);
#15213=ORIENTED_EDGE('',*,*,#11115,.F.);
#15214=ORIENTED_EDGE('',*,*,#11118,.T.);
#15215=ORIENTED_EDGE('',*,*,#11192,.T.);
#15216=ORIENTED_EDGE('',*,*,#11177,.T.);
#15217=ORIENTED_EDGE('',*,*,#11121,.F.);
#15218=ORIENTED_EDGE('',*,*,#11125,.T.);
#15219=ORIENTED_EDGE('',*,*,#11128,.F.);
#15220=ORIENTED_EDGE('',*,*,#11131,.T.);
#15221=ORIENTED_EDGE('',*,*,#11193,.T.);
#15222=ORIENTED_EDGE('',*,*,#11194,.T.);
#15223=ORIENTED_EDGE('',*,*,#11134,.F.);
#15224=ORIENTED_EDGE('',*,*,#11138,.T.);
#15225=ORIENTED_EDGE('',*,*,#11141,.F.);
#15226=ORIENTED_EDGE('',*,*,#11144,.T.);
#15227=ORIENTED_EDGE('',*,*,#11186,.T.);
#15228=ORIENTED_EDGE('',*,*,#11174,.T.);
#15229=ORIENTED_EDGE('',*,*,#11147,.F.);
#15230=ORIENTED_EDGE('',*,*,#11151,.T.);
#15231=ORIENTED_EDGE('',*,*,#11154,.F.);
#15232=ORIENTED_EDGE('',*,*,#11157,.T.);
#15233=ORIENTED_EDGE('',*,*,#11195,.T.);
#15234=ORIENTED_EDGE('',*,*,#11130,.T.);
#15235=ORIENTED_EDGE('',*,*,#11196,.F.);
#15236=ORIENTED_EDGE('',*,*,#11197,.T.);
#15237=ORIENTED_EDGE('',*,*,#11193,.F.);
#15238=ORIENTED_EDGE('',*,*,#11181,.T.);
#15239=ORIENTED_EDGE('',*,*,#11191,.F.);
#15240=ORIENTED_EDGE('',*,*,#11198,.T.);
#15241=ORIENTED_EDGE('',*,*,#11199,.F.);
#15242=ORIENTED_EDGE('',*,*,#11135,.F.);
#15243=ORIENTED_EDGE('',*,*,#11194,.F.);
#15244=ORIENTED_EDGE('',*,*,#11197,.F.);
#15245=ORIENTED_EDGE('',*,*,#11200,.F.);
#15246=ORIENTED_EDGE('',*,*,#11172,.T.);
#15247=ORIENTED_EDGE('',*,*,#11195,.F.);
#15248=ORIENTED_EDGE('',*,*,#11156,.T.);
#15249=ORIENTED_EDGE('',*,*,#11201,.F.);
#15250=ORIENTED_EDGE('',*,*,#11184,.F.);
#15251=ORIENTED_EDGE('',*,*,#11202,.F.);
#15252=ORIENTED_EDGE('',*,*,#11203,.F.);
#15253=ORIENTED_EDGE('',*,*,#11188,.F.);
#15254=ORIENTED_EDGE('',*,*,#11203,.T.);
#15255=ORIENTED_EDGE('',*,*,#11204,.F.);
#15256=ORIENTED_EDGE('',*,*,#11205,.F.);
#15257=ORIENTED_EDGE('',*,*,#11189,.F.);
#15258=ORIENTED_EDGE('',*,*,#11205,.T.);
#15259=ORIENTED_EDGE('',*,*,#11206,.F.);
#15260=ORIENTED_EDGE('',*,*,#11198,.F.);
#15261=ORIENTED_EDGE('',*,*,#11190,.F.);
#15262=ORIENTED_EDGE('',*,*,#11178,.T.);
#15263=ORIENTED_EDGE('',*,*,#11192,.F.);
#15264=ORIENTED_EDGE('',*,*,#11117,.T.);
#15265=ORIENTED_EDGE('',*,*,#11207,.F.);
#15266=ORIENTED_EDGE('',*,*,#11173,.T.);
#15267=ORIENTED_EDGE('',*,*,#11201,.T.);
#15268=ORIENTED_EDGE('',*,*,#11155,.T.);
#15269=ORIENTED_EDGE('',*,*,#11152,.F.);
#15270=ORIENTED_EDGE('',*,*,#11149,.T.);
#15271=ORIENTED_EDGE('',*,*,#11145,.F.);
#15272=ORIENTED_EDGE('',*,*,#11176,.T.);
#15273=ORIENTED_EDGE('',*,*,#11187,.T.);
#15274=ORIENTED_EDGE('',*,*,#11142,.T.);
#15275=ORIENTED_EDGE('',*,*,#11139,.F.);
#15276=ORIENTED_EDGE('',*,*,#11136,.T.);
#15277=ORIENTED_EDGE('',*,*,#11132,.F.);
#15278=ORIENTED_EDGE('',*,*,#11200,.T.);
#15279=ORIENTED_EDGE('',*,*,#11196,.T.);
#15280=ORIENTED_EDGE('',*,*,#11129,.T.);
#15281=ORIENTED_EDGE('',*,*,#11126,.F.);
#15282=ORIENTED_EDGE('',*,*,#11123,.T.);
#15283=ORIENTED_EDGE('',*,*,#11119,.F.);
#15284=ORIENTED_EDGE('',*,*,#11179,.T.);
#15285=ORIENTED_EDGE('',*,*,#11207,.T.);
#15286=ORIENTED_EDGE('',*,*,#11116,.T.);
#15287=ORIENTED_EDGE('',*,*,#11113,.F.);
#15288=ORIENTED_EDGE('',*,*,#11110,.T.);
#15289=ORIENTED_EDGE('',*,*,#11106,.F.);
#15290=ORIENTED_EDGE('',*,*,#11182,.T.);
#15291=ORIENTED_EDGE('',*,*,#11199,.T.);
#15292=ORIENTED_EDGE('',*,*,#11206,.T.);
#15293=ORIENTED_EDGE('',*,*,#11204,.T.);
#15294=ORIENTED_EDGE('',*,*,#11202,.T.);
#15295=ORIENTED_EDGE('',*,*,#11183,.T.);
#15296=ORIENTED_EDGE('',*,*,#11168,.T.);
#15297=ORIENTED_EDGE('',*,*,#11165,.F.);
#15298=ORIENTED_EDGE('',*,*,#11162,.T.);
#15299=ORIENTED_EDGE('',*,*,#11158,.F.);
#18932=ADVANCED_FACE('',(#5216),#4482,.F.);
#18933=ADVANCED_FACE('',(#5217),#4483,.F.);
#18934=ADVANCED_FACE('',(#5218),#4484,.F.);
#18935=ADVANCED_FACE('',(#5219),#802,.F.);
#18936=ADVANCED_FACE('',(#5220),#4485,.F.);
#18937=ADVANCED_FACE('',(#5221),#4486,.F.);
#18938=ADVANCED_FACE('',(#5222),#4487,.F.);
#18939=ADVANCED_FACE('',(#5223),#803,.F.);
#18940=ADVANCED_FACE('',(#5224),#4488,.F.);
#18941=ADVANCED_FACE('',(#5225),#4489,.F.);
#18942=ADVANCED_FACE('',(#5226),#4490,.F.);
#18943=ADVANCED_FACE('',(#5227),#804,.F.);
#18944=ADVANCED_FACE('',(#5228),#4491,.F.);
#18945=ADVANCED_FACE('',(#5229),#4492,.F.);
#18946=ADVANCED_FACE('',(#5230),#4493,.F.);
#18947=ADVANCED_FACE('',(#5231),#805,.F.);
#18948=ADVANCED_FACE('',(#5232),#4494,.F.);
#18949=ADVANCED_FACE('',(#5233),#4495,.F.);
#18950=ADVANCED_FACE('',(#5234),#4496,.F.);
#18951=ADVANCED_FACE('',(#5235),#806,.F.);
#18952=ADVANCED_FACE('',(#5236),#807,.F.);
#18953=ADVANCED_FACE('',(#5237),#808,.F.);
#18954=ADVANCED_FACE('',(#5238),#809,.F.);
#18955=ADVANCED_FACE('',(#5239),#810,.F.);
#18956=ADVANCED_FACE('',(#5240),#4497,.F.);
#18957=ADVANCED_FACE('',(#5241),#4498,.F.);
#18958=ADVANCED_FACE('',(#5242),#811,.F.);
#18959=ADVANCED_FACE('',(#5243),#4499,.F.);
#18960=ADVANCED_FACE('',(#5244),#4500,.F.);
#18961=ADVANCED_FACE('',(#5245),#812,.F.);
#18962=ADVANCED_FACE('',(#5246),#4501,.F.);
#18963=ADVANCED_FACE('',(#5247),#813,.T.);
#18964=ADVANCED_FACE('',(#5248),#4502,.T.);
#18965=ADVANCED_FACE('',(#5249),#814,.T.);
#18966=ADVANCED_FACE('',(#5250),#4503,.F.);
#18967=ADVANCED_FACE('',(#5251),#815,.T.);
#19564=CLOSED_SHELL('',(#18932,#18933,#18934,#18935,#18936,#18937,#18938,
#18939,#18940,#18941,#18942,#18943,#18944,#18945,#18946,#18947,#18948,#18949,
#18950,#18951,#18952,#18953,#18954,#18955,#18956,#18957,#18958,#18959,#18960,
#18961,#18962,#18963,#18964,#18965,#18966,#18967));
#20884=AXIS2_PLACEMENT_3D('',#31101,#24750,#24751);
#20885=AXIS2_PLACEMENT_3D('',#31102,#24752,#24753);
#20886=AXIS2_PLACEMENT_3D('',#31105,#24754,#24755);
#20887=AXIS2_PLACEMENT_3D('',#31109,#24757,#24758);
#20888=AXIS2_PLACEMENT_3D('',#31111,#24760,#24761);
#20889=AXIS2_PLACEMENT_3D('',#31113,#24762,#24763);
#20890=AXIS2_PLACEMENT_3D('',#31116,#24765,#24766);
#20891=AXIS2_PLACEMENT_3D('',#31117,#24767,#24768);
#20892=AXIS2_PLACEMENT_3D('',#31119,#24769,#24770);
#20893=AXIS2_PLACEMENT_3D('',#31122,#24772,#24773);
#20894=AXIS2_PLACEMENT_3D('',#31123,#24774,#24775);
#20895=AXIS2_PLACEMENT_3D('',#31129,#24779,#24780);
#20896=AXIS2_PLACEMENT_3D('',#31132,#24781,#24782);
#20897=AXIS2_PLACEMENT_3D('',#31136,#24784,#24785);
#20898=AXIS2_PLACEMENT_3D('',#31138,#24787,#24788);
#20899=AXIS2_PLACEMENT_3D('',#31140,#24789,#24790);
#20900=AXIS2_PLACEMENT_3D('',#31143,#24792,#24793);
#20901=AXIS2_PLACEMENT_3D('',#31144,#24794,#24795);
#20902=AXIS2_PLACEMENT_3D('',#31146,#24796,#24797);
#20903=AXIS2_PLACEMENT_3D('',#31149,#24799,#24800);
#20904=AXIS2_PLACEMENT_3D('',#31150,#24801,#24802);
#20905=AXIS2_PLACEMENT_3D('',#31156,#24806,#24807);
#20906=AXIS2_PLACEMENT_3D('',#31159,#24808,#24809);
#20907=AXIS2_PLACEMENT_3D('',#31163,#24811,#24812);
#20908=AXIS2_PLACEMENT_3D('',#31165,#24814,#24815);
#20909=AXIS2_PLACEMENT_3D('',#31167,#24816,#24817);
#20910=AXIS2_PLACEMENT_3D('',#31170,#24819,#24820);
#20911=AXIS2_PLACEMENT_3D('',#31171,#24821,#24822);
#20912=AXIS2_PLACEMENT_3D('',#31173,#24823,#24824);
#20913=AXIS2_PLACEMENT_3D('',#31176,#24826,#24827);
#20914=AXIS2_PLACEMENT_3D('',#31177,#24828,#24829);
#20915=AXIS2_PLACEMENT_3D('',#31183,#24833,#24834);
#20916=AXIS2_PLACEMENT_3D('',#31186,#24835,#24836);
#20917=AXIS2_PLACEMENT_3D('',#31190,#24838,#24839);
#20918=AXIS2_PLACEMENT_3D('',#31192,#24841,#24842);
#20919=AXIS2_PLACEMENT_3D('',#31194,#24843,#24844);
#20920=AXIS2_PLACEMENT_3D('',#31197,#24846,#24847);
#20921=AXIS2_PLACEMENT_3D('',#31198,#24848,#24849);
#20922=AXIS2_PLACEMENT_3D('',#31200,#24850,#24851);
#20923=AXIS2_PLACEMENT_3D('',#31203,#24853,#24854);
#20924=AXIS2_PLACEMENT_3D('',#31204,#24855,#24856);
#20925=AXIS2_PLACEMENT_3D('',#31210,#24860,#24861);
#20926=AXIS2_PLACEMENT_3D('',#31213,#24862,#24863);
#20927=AXIS2_PLACEMENT_3D('',#31217,#24865,#24866);
#20928=AXIS2_PLACEMENT_3D('',#31219,#24868,#24869);
#20929=AXIS2_PLACEMENT_3D('',#31221,#24870,#24871);
#20930=AXIS2_PLACEMENT_3D('',#31224,#24873,#24874);
#20931=AXIS2_PLACEMENT_3D('',#31225,#24875,#24876);
#20932=AXIS2_PLACEMENT_3D('',#31227,#24877,#24878);
#20933=AXIS2_PLACEMENT_3D('',#31230,#24880,#24881);
#20934=AXIS2_PLACEMENT_3D('',#31231,#24882,#24883);
#20935=AXIS2_PLACEMENT_3D('',#31237,#24887,#24888);
#20936=AXIS2_PLACEMENT_3D('',#31243,#24892,#24893);
#20937=AXIS2_PLACEMENT_3D('',#31249,#24897,#24898);
#20938=AXIS2_PLACEMENT_3D('',#31255,#24902,#24903);
#20939=AXIS2_PLACEMENT_3D('',#31261,#24907,#24908);
#20940=AXIS2_PLACEMENT_3D('',#31263,#24909,#24910);
#20941=AXIS2_PLACEMENT_3D('',#31266,#24912,#24913);
#20942=AXIS2_PLACEMENT_3D('',#31267,#24914,#24915);
#20943=AXIS2_PLACEMENT_3D('',#31268,#24916,#24917);
#20944=AXIS2_PLACEMENT_3D('',#31269,#24918,#24919);
#20945=AXIS2_PLACEMENT_3D('',#31270,#24920,#24921);
#20946=AXIS2_PLACEMENT_3D('',#31274,#24923,#24924);
#20947=AXIS2_PLACEMENT_3D('',#31277,#24926,#24927);
#20948=AXIS2_PLACEMENT_3D('',#31278,#24928,#24929);
#20949=AXIS2_PLACEMENT_3D('',#31280,#24930,#24931);
#20950=AXIS2_PLACEMENT_3D('',#31282,#24933,#24934);
#20951=AXIS2_PLACEMENT_3D('',#31283,#24935,#24936);
#20952=AXIS2_PLACEMENT_3D('',#31285,#24937,#24938);
#20953=AXIS2_PLACEMENT_3D('',#31287,#24940,#24941);
#20954=AXIS2_PLACEMENT_3D('',#31290,#24943,#24944);
#20955=AXIS2_PLACEMENT_3D('',#31291,#24945,#24946);
#20956=AXIS2_PLACEMENT_3D('',#31293,#24948,#24949);
#20957=AXIS2_PLACEMENT_3D('',#31294,#24950,#24951);
#20958=AXIS2_PLACEMENT_3D('',#31295,#24952,#24953);
#20959=AXIS2_PLACEMENT_3D('',#31299,#24956,#24957);
#20960=AXIS2_PLACEMENT_3D('',#31301,#24958,#24959);
#20961=AXIS2_PLACEMENT_3D('',#31303,#24961,#24962);
#20962=AXIS2_PLACEMENT_3D('',#31305,#24964,#24965);
#20963=AXIS2_PLACEMENT_3D('',#31306,#24966,#24967);
#20964=AXIS2_PLACEMENT_3D('',#31307,#24968,#24969);
#24750=DIRECTION('axis',(0.,0.,1.));
#24751=DIRECTION('refdir',(1.,0.,0.));
#24752=DIRECTION('center_axis',(0.,-1.,0.));
#24753=DIRECTION('ref_axis',(0.877771605587211,0.,-0.479079334165908));
#24754=DIRECTION('center_axis',(0.,1.,0.));
#24755=DIRECTION('ref_axis',(0.877771605579571,0.,-0.479079334179906));
#24756=DIRECTION('',(0.,-1.,0.));
#24757=DIRECTION('center_axis',(0.,-1.,0.));
#24758=DIRECTION('ref_axis',(0.877771605579571,0.,-0.479079334179906));
#24759=DIRECTION('',(0.,1.,0.));
#24760=DIRECTION('center_axis',(0.,-1.,0.));
#24761=DIRECTION('ref_axis',(0.290991366091359,0.,-0.956725679001188));
#24762=DIRECTION('center_axis',(0.,-1.,0.));
#24763=DIRECTION('ref_axis',(0.290991366091832,0.,-0.956725679001044));
#24764=DIRECTION('',(0.,1.,0.));
#24765=DIRECTION('center_axis',(0.,1.,0.));
#24766=DIRECTION('ref_axis',(0.290991366091832,0.,-0.956725679001044));
#24767=DIRECTION('center_axis',(0.,-1.,0.));
#24768=DIRECTION('ref_axis',(-0.520632842076221,0.,-0.853780676609419));
#24769=DIRECTION('center_axis',(0.,1.,0.));
#24770=DIRECTION('ref_axis',(-0.520632842087598,0.,-0.853780676602481));
#24771=DIRECTION('',(0.,-1.,0.));
#24772=DIRECTION('center_axis',(0.,-1.,0.));
#24773=DIRECTION('ref_axis',(-0.520632842087598,0.,-0.853780676602481));
#24774=DIRECTION('center_axis',(-0.974044425513625,0.,-0.22635692418354));
#24775=DIRECTION('ref_axis',(-0.22635692418354,0.,0.974044425513625));
#24776=DIRECTION('',(0.226356924184268,0.,-0.974044425513455));
#24777=DIRECTION('',(0.,1.,0.));
#24778=DIRECTION('',(-0.226356924184268,0.,0.974044425513455));
#24779=DIRECTION('center_axis',(0.,-1.,0.));
#24780=DIRECTION('ref_axis',(0.80772974655928,0.,-0.589552929365364));
#24781=DIRECTION('center_axis',(0.,1.,0.));
#24782=DIRECTION('ref_axis',(0.807729746554134,0.,-0.589552929372413));
#24783=DIRECTION('',(0.,-1.,0.));
#24784=DIRECTION('center_axis',(0.,-1.,0.));
#24785=DIRECTION('ref_axis',(0.807729746554134,0.,-0.589552929372413));
#24786=DIRECTION('',(0.,1.,0.));
#24787=DIRECTION('center_axis',(0.,-1.,0.));
#24788=DIRECTION('ref_axis',(0.163624134736254,0.,-0.986522753174914));
#24789=DIRECTION('center_axis',(0.,-1.,0.));
#24790=DIRECTION('ref_axis',(0.163624134736857,0.,-0.986522753174814));
#24791=DIRECTION('',(0.,1.,0.));
#24792=DIRECTION('center_axis',(0.,1.,0.));
#24793=DIRECTION('ref_axis',(0.163624134736857,0.,-0.986522753174814));
#24794=DIRECTION('center_axis',(0.,-1.,0.));
#24795=DIRECTION('ref_axis',(-0.627619496647803,0.,-0.778520242143747));
#24796=DIRECTION('center_axis',(0.,1.,0.));
#24797=DIRECTION('ref_axis',(-0.627619496652502,0.,-0.778520242139959));
#24798=DIRECTION('',(0.,-1.,0.));
#24799=DIRECTION('center_axis',(0.,-1.,0.));
#24800=DIRECTION('ref_axis',(-0.627619496652502,0.,-0.778520242139959));
#24801=DIRECTION('center_axis',(-0.995256847821609,0.,-0.0972820994026906));
#24802=DIRECTION('ref_axis',(-0.0972820994026906,0.,0.995256847821609));
#24803=DIRECTION('',(0.0972820994035842,0.,-0.995256847821521));
#24804=DIRECTION('',(0.,1.,0.));
#24805=DIRECTION('',(-0.0972820994035842,0.,0.995256847821521));
#24806=DIRECTION('center_axis',(0.,-1.,0.));
#24807=DIRECTION('ref_axis',(0.723867407622732,0.,-0.689939110488415));
#24808=DIRECTION('center_axis',(0.,1.,0.));
#24809=DIRECTION('ref_axis',(0.723867407621795,0.,-0.689939110489398));
#24810=DIRECTION('',(0.,-1.,0.));
#24811=DIRECTION('center_axis',(0.,-1.,0.));
#24812=DIRECTION('ref_axis',(0.723867407621795,0.,-0.689939110489398));
#24813=DIRECTION('',(0.,1.,0.));
#24814=DIRECTION('center_axis',(0.,-1.,0.));
#24815=DIRECTION('ref_axis',(0.0334572490706318,0.,-0.999440149526036));
#24816=DIRECTION('center_axis',(0.,-1.,0.));
#24817=DIRECTION('ref_axis',(0.0334572490713496,0.,-0.999440149526012));
#24818=DIRECTION('',(0.,1.,0.));
#24819=DIRECTION('center_axis',(0.,1.,0.));
#24820=DIRECTION('ref_axis',(0.0334572490713496,0.,-0.999440149526012));
#24821=DIRECTION('center_axis',(0.,-1.,0.));
#24822=DIRECTION('ref_axis',(-0.723867407622738,0.,-0.689939110488409));
#24823=DIRECTION('center_axis',(0.,1.,0.));
#24824=DIRECTION('ref_axis',(-0.723867407621802,0.,-0.689939110489391));
#24825=DIRECTION('',(0.,-1.,0.));
#24826=DIRECTION('center_axis',(0.,-1.,0.));
#24827=DIRECTION('ref_axis',(-0.723867407621802,0.,-0.689939110489391));
#24828=DIRECTION('center_axis',(-0.999440149526036,0.,0.0334572490706321));
#24829=DIRECTION('ref_axis',(0.,1.,0.));
#24830=DIRECTION('',(-0.0334572490715975,0.,-0.999440149526004));
#24831=DIRECTION('',(0.,1.,0.));
#24832=DIRECTION('',(0.0334572490715975,0.,0.999440149526004));
#24833=DIRECTION('center_axis',(0.,-1.,0.));
#24834=DIRECTION('ref_axis',(0.627619496647802,0.,-0.778520242143748));
#24835=DIRECTION('center_axis',(0.,1.,0.));
#24836=DIRECTION('ref_axis',(0.627619496652501,0.,-0.77852024213996));
#24837=DIRECTION('',(0.,-1.,0.));
#24838=DIRECTION('center_axis',(0.,-1.,0.));
#24839=DIRECTION('ref_axis',(0.627619496652501,0.,-0.77852024213996));
#24840=DIRECTION('',(0.,1.,0.));
#24841=DIRECTION('center_axis',(0.,-1.,0.));
#24842=DIRECTION('ref_axis',(-0.097282099402691,0.,-0.995256847821609));
#24843=DIRECTION('center_axis',(0.,-1.,0.));
#24844=DIRECTION('ref_axis',(-0.0972820994033555,0.,-0.995256847821544));
#24845=DIRECTION('',(0.,1.,0.));
#24846=DIRECTION('center_axis',(0.,1.,0.));
#24847=DIRECTION('ref_axis',(-0.0972820994033555,0.,-0.995256847821544));
#24848=DIRECTION('center_axis',(0.,-1.,0.));
#24849=DIRECTION('ref_axis',(-0.807729746559285,0.,-0.589552929365357));
#24850=DIRECTION('center_axis',(0.,1.,0.));
#24851=DIRECTION('ref_axis',(-0.80772974655414,0.,-0.589552929372406));
#24852=DIRECTION('',(0.,-1.,0.));
#24853=DIRECTION('center_axis',(0.,-1.,0.));
#24854=DIRECTION('ref_axis',(-0.80772974655414,0.,-0.589552929372406));
#24855=DIRECTION('center_axis',(-0.986522753174914,0.,0.163624134736254));
#24856=DIRECTION('ref_axis',(0.,1.,0.));
#24857=DIRECTION('',(-0.163624134737066,0.,-0.986522753174779));
#24858=DIRECTION('',(0.,1.,0.));
#24859=DIRECTION('',(0.163624134737066,0.,0.986522753174779));
#24860=DIRECTION('center_axis',(0.,-1.,0.));
#24861=DIRECTION('ref_axis',(0.520632842076226,0.,-0.853780676609416));
#24862=DIRECTION('center_axis',(0.,1.,0.));
#24863=DIRECTION('ref_axis',(0.520632842087603,0.,-0.853780676602478));
#24864=DIRECTION('',(0.,-1.,0.));
#24865=DIRECTION('center_axis',(0.,-1.,0.));
#24866=DIRECTION('ref_axis',(0.520632842087603,0.,-0.853780676602478));
#24867=DIRECTION('',(0.,1.,0.));
#24868=DIRECTION('center_axis',(0.,-1.,0.));
#24869=DIRECTION('ref_axis',(-0.22635692418354,0.,-0.974044425513625));
#24870=DIRECTION('center_axis',(0.,-1.,0.));
#24871=DIRECTION('ref_axis',(-0.226356924184081,0.,-0.974044425513499));
#24872=DIRECTION('',(0.,1.,0.));
#24873=DIRECTION('center_axis',(0.,1.,0.));
#24874=DIRECTION('ref_axis',(-0.226356924184081,0.,-0.974044425513499));
#24875=DIRECTION('center_axis',(0.,-1.,0.));
#24876=DIRECTION('ref_axis',(-0.877771605587215,0.,-0.4790793341659));
#24877=DIRECTION('center_axis',(0.,1.,0.));
#24878=DIRECTION('ref_axis',(-0.877771605579575,0.,-0.479079334179899));
#24879=DIRECTION('',(0.,-1.,0.));
#24880=DIRECTION('center_axis',(0.,-1.,0.));
#24881=DIRECTION('ref_axis',(-0.877771605579575,0.,-0.479079334179899));
#24882=DIRECTION('center_axis',(-0.956725679001188,0.,0.290991366091359));
#24883=DIRECTION('ref_axis',(0.,1.,0.));
#24884=DIRECTION('',(-0.290991366091996,0.,-0.956725679000994));
#24885=DIRECTION('',(0.,1.,0.));
#24886=DIRECTION('',(0.290991366091996,0.,0.956725679000994));
#24887=DIRECTION('center_axis',(0.974044425513625,0.,-0.22635692418354));
#24888=DIRECTION('ref_axis',(0.,-1.,0.));
#24889=DIRECTION('',(-0.226356924184268,0.,-0.974044425513455));
#24890=DIRECTION('',(0.,-1.,0.));
#24891=DIRECTION('',(0.226356924184268,0.,0.974044425513455));
#24892=DIRECTION('center_axis',(0.995256847821609,0.,-0.0972820994026909));
#24893=DIRECTION('ref_axis',(0.,-1.,0.));
#24894=DIRECTION('',(-0.0972820994035846,0.,-0.995256847821521));
#24895=DIRECTION('',(0.,-1.,0.));
#24896=DIRECTION('',(0.0972820994035846,0.,0.995256847821521));
#24897=DIRECTION('center_axis',(0.986522753174914,0.,0.163624134736254));
#24898=DIRECTION('ref_axis',(0.,-1.,0.));
#24899=DIRECTION('',(0.163624134737066,0.,-0.986522753174779));
#24900=DIRECTION('',(0.,-1.,0.));
#24901=DIRECTION('',(-0.163624134737066,0.,0.986522753174779));
#24902=DIRECTION('center_axis',(0.956725679001189,0.,0.290991366091358));
#24903=DIRECTION('ref_axis',(0.,-1.,0.));
#24904=DIRECTION('',(0.290991366091995,0.,-0.956725679000995));
#24905=DIRECTION('',(0.,-1.,0.));
#24906=DIRECTION('',(-0.290991366091995,0.,0.956725679000995));
#24907=DIRECTION('center_axis',(0.,1.,0.));
#24908=DIRECTION('ref_axis',(-0.333806859233771,0.,0.942641491092178));
#24909=DIRECTION('center_axis',(0.,-1.,0.));
#24910=DIRECTION('ref_axis',(-0.333806859234212,0.,0.942641491092022));
#24911=DIRECTION('',(0.,-1.,0.));
#24912=DIRECTION('center_axis',(0.,1.,0.));
#24913=DIRECTION('ref_axis',(-0.333806859234212,0.,0.942641491092022));
#24914=DIRECTION('center_axis',(0.,1.,0.));
#24915=DIRECTION('ref_axis',(-0.333806859233771,0.,0.942641491092178));
#24916=DIRECTION('center_axis',(0.,1.,0.));
#24917=DIRECTION('ref_axis',(-0.333806859234212,0.,0.942641491092022));
#24918=DIRECTION('center_axis',(0.,-1.,0.));
#24919=DIRECTION('ref_axis',(-0.333806859234212,0.,0.942641491092022));
#24920=DIRECTION('center_axis',(0.,1.,0.));
#24921=DIRECTION('ref_axis',(1.,0.,0.));
#24922=DIRECTION('',(-0.333806859234348,0.,-0.942641491091974));
#24923=DIRECTION('center_axis',(0.,-1.,0.));
#24924=DIRECTION('ref_axis',(0.333806859234184,0.,-0.942641491092032));
#24925=DIRECTION('',(-0.333806859234344,0.,0.942641491091975));
#24926=DIRECTION('center_axis',(0.,1.,0.));
#24927=DIRECTION('ref_axis',(-0.333806859234212,0.,0.942641491092022));
#24928=DIRECTION('center_axis',(0.,1.,0.));
#24929=DIRECTION('ref_axis',(-0.333806859234212,0.,0.942641491092022));
#24930=DIRECTION('center_axis',(0.,1.,0.));
#24931=DIRECTION('ref_axis',(-0.333806859234212,0.,0.942641491092022));
#24932=DIRECTION('',(0.0334572490715973,0.,-0.999440149526004));
#24933=DIRECTION('center_axis',(0.,1.,0.));
#24934=DIRECTION('ref_axis',(-0.333806859234212,0.,0.942641491092022));
#24935=DIRECTION('center_axis',(0.,1.,0.));
#24936=DIRECTION('ref_axis',(-0.333806859233771,0.,0.942641491092178));
#24937=DIRECTION('center_axis',(0.,-1.,0.));
#24938=DIRECTION('ref_axis',(-0.333806859234212,0.,0.942641491092022));
#24939=DIRECTION('',(0.,-1.,0.));
#24940=DIRECTION('center_axis',(0.,1.,0.));
#24941=DIRECTION('ref_axis',(-0.333806859233771,0.,0.942641491092178));
#24942=DIRECTION('',(0.,1.,0.));
#24943=DIRECTION('center_axis',(0.,-1.,0.));
#24944=DIRECTION('ref_axis',(-0.333806859234212,0.,0.942641491092022));
#24945=DIRECTION('center_axis',(0.999440149526036,0.,0.0334572490706318));
#24946=DIRECTION('ref_axis',(0.,-1.,0.));
#24947=DIRECTION('',(-0.0334572490715973,0.,0.999440149526004));
#24948=DIRECTION('center_axis',(0.,1.,0.));
#24949=DIRECTION('ref_axis',(-0.333806859233771,0.,0.942641491092178));
#24950=DIRECTION('center_axis',(0.,-1.,0.));
#24951=DIRECTION('ref_axis',(-0.333806859234212,0.,0.942641491092022));
#24952=DIRECTION('center_axis',(-0.942641491092177,0.,0.333806859233774));
#24953=DIRECTION('ref_axis',(0.,1.,0.));
#24954=DIRECTION('',(0.333806859234348,0.,0.942641491091974));
#24955=DIRECTION('',(0.,1.,0.));
#24956=DIRECTION('center_axis',(0.,1.,0.));
#24957=DIRECTION('ref_axis',(0.333806859233771,0.,-0.942641491092178));
#24958=DIRECTION('center_axis',(0.,1.,0.));
#24959=DIRECTION('ref_axis',(0.333806859234184,0.,-0.942641491092032));
#24960=DIRECTION('',(0.,1.,0.));
#24961=DIRECTION('center_axis',(0.942641491092179,0.,0.33380685923377));
#24962=DIRECTION('ref_axis',(0.,-1.,0.));
#24963=DIRECTION('',(0.333806859234344,0.,-0.942641491091975));
#24964=DIRECTION('center_axis',(0.,1.,0.));
#24965=DIRECTION('ref_axis',(-0.333806859233771,0.,0.942641491092178));
#24966=DIRECTION('center_axis',(0.,-1.,0.));
#24967=DIRECTION('ref_axis',(-0.333806859234212,0.,0.942641491092022));
#24968=DIRECTION('center_axis',(0.,1.,0.));
#24969=DIRECTION('ref_axis',(1.,0.,0.));
#31101=CARTESIAN_POINT('',(0.,0.,0.));
#31102=CARTESIAN_POINT('Origin',(0.00360121565085287,-0.008,-0.0126992616256242));
#31103=CARTESIAN_POINT('',(0.00384039707060316,-0.008,-0.0126265137841014));
#31104=CARTESIAN_POINT('',(0.00366942049272508,-0.008,-0.0129397779442914));
#31105=CARTESIAN_POINT('Origin',(0.00360121565086286,-0.00799999999999,
-0.0126992616256342));
#31106=CARTESIAN_POINT('',(0.00366942049272508,-0.024,-0.0129397779442914));
#31107=CARTESIAN_POINT('',(0.00366942049273508,-0.00799999999999,-0.0129397779443014));
#31108=CARTESIAN_POINT('',(0.00384039707060316,-0.024,-0.0126265137841014));
#31109=CARTESIAN_POINT('Origin',(0.00360121565086286,-0.02400000000001,
-0.0126992616256342));
#31110=CARTESIAN_POINT('',(0.00384039707061316,-0.00799999999999,-0.0126265137841114));
#31111=CARTESIAN_POINT('Origin',(-4.44089209850063E-17,-0.008,6.72997231505748E-33));
#31112=CARTESIAN_POINT('',(0.00329207760827845,-0.008,-0.0130408866654485));
#31113=CARTESIAN_POINT('Origin',(-4.44089209850063E-17,-0.00799999999999,
6.72997231505748E-33));
#31114=CARTESIAN_POINT('',(0.00329207760827845,-0.024,-0.0130408866654485));
#31115=CARTESIAN_POINT('',(0.00329207760828845,-0.00799999999999,-0.0130408866654585));
#31116=CARTESIAN_POINT('Origin',(-4.44089209850063E-17,-0.02400000000001,
6.72997231505748E-33));
#31117=CARTESIAN_POINT('Origin',(0.00323088657466734,-0.008,-0.0127984910025219));
#31118=CARTESIAN_POINT('',(0.00298737546828893,-0.008,-0.0128550802335678));
#31119=CARTESIAN_POINT('Origin',(0.00323088657467733,-0.00799999999999,
-0.0127984910025319));
#31120=CARTESIAN_POINT('',(0.00298737546828893,-0.024,-0.0128550802335678));
#31121=CARTESIAN_POINT('',(0.00298737546829892,-0.00799999999999,-0.0128550802335778));
#31122=CARTESIAN_POINT('Origin',(0.00323088657467733,-0.02400000000001,
-0.0127984910025319));
#31123=CARTESIAN_POINT('Origin',(0.00294264001438597,-0.008,-0.0126625775316771));
#31124=CARTESIAN_POINT('',(0.00294264001438597,-0.008,-0.0126625775316771));
#31125=CARTESIAN_POINT('',(0.00291295831081407,-0.00799999999999,-0.0125348531511851));
#31126=CARTESIAN_POINT('',(0.00294264001438597,-0.024,-0.0126625775316771));
#31127=CARTESIAN_POINT('',(0.00294264001439597,-0.016,-0.0126625775316871));
#31128=CARTESIAN_POINT('',(0.00291295831081407,-0.02400000000001,-0.0125348531511851));
#31129=CARTESIAN_POINT('Origin',(0.00191282048773806,-0.008,-0.0130606706482359));
#31130=CARTESIAN_POINT('',(0.00215945117603179,-0.008,-0.0130197646145518));
#31131=CARTESIAN_POINT('',(0.00194904814849068,-0.008,-0.0133080318347555));
#31132=CARTESIAN_POINT('Origin',(0.00191282048774806,-0.00799999999999,
-0.0130606706482459));
#31133=CARTESIAN_POINT('',(0.00194904814849068,-0.024,-0.0133080318347555));
#31134=CARTESIAN_POINT('',(0.00194904814850068,-0.00799999999999,-0.0133080318347655));
#31135=CARTESIAN_POINT('',(0.00215945117603179,-0.024,-0.0130197646145518));
#31136=CARTESIAN_POINT('Origin',(0.00191282048774806,-0.02400000000001,
-0.0130606706482459));
#31137=CARTESIAN_POINT('',(0.0021594511760418,-0.00799999999999,-0.0130197646145618));
#31138=CARTESIAN_POINT('Origin',(-4.44089209850063E-17,-0.008,6.72997231505748E-33));
#31139=CARTESIAN_POINT('',(0.00156173614835723,-0.008,-0.0133590224269186));
#31140=CARTESIAN_POINT('Origin',(-4.44089209850063E-17,-0.00799999999999,
6.72997231505748E-33));
#31141=CARTESIAN_POINT('',(0.00156173614835723,-0.024,-0.0133590224269186));
#31142=CARTESIAN_POINT('',(0.00156173614836722,-0.00799999999999,-0.0133590224269286));
#31143=CARTESIAN_POINT('Origin',(-4.44089209850063E-17,-0.02400000000001,
6.72997231505748E-33));
#31144=CARTESIAN_POINT('Origin',(0.00153270759541378,-0.008,-0.0131107134598755));
#31145=CARTESIAN_POINT('',(0.00128389338345838,-0.008,-0.0131350339847262));
#31146=CARTESIAN_POINT('Origin',(0.00153270759542378,-0.00799999999999,
-0.0131107134598855));
#31147=CARTESIAN_POINT('',(0.00128389338345838,-0.024,-0.0131350339847262));
#31148=CARTESIAN_POINT('',(0.00128389338346838,-0.00799999999999,-0.0131350339847362));
#31149=CARTESIAN_POINT('Origin',(0.00153270759542378,-0.02400000000001,
-0.0131107134598855));
#31150=CARTESIAN_POINT('Origin',(0.00126466729223494,-0.008,-0.0129383390216809));
#31151=CARTESIAN_POINT('',(0.00126466729223494,-0.008,-0.0129383390216809));
#31152=CARTESIAN_POINT('',(0.00126540384839637,-0.00799999999999,-0.0129458744527519));
#31153=CARTESIAN_POINT('',(0.00126466729223494,-0.024,-0.0129383390216809));
#31154=CARTESIAN_POINT('',(0.00126466729224494,-0.016,-0.0129383390216909));
#31155=CARTESIAN_POINT('',(0.00126540384839637,-0.02400000000001,-0.0129458744527519));
#31156=CARTESIAN_POINT('Origin',(0.000191696435744033,-0.008,-0.0131986079749541));
#31157=CARTESIAN_POINT('',(0.000441556473125542,-0.008,-0.0131902436626865));
#31158=CARTESIAN_POINT('',(0.000195327050057368,-0.008,-0.0134485816108434));
#31159=CARTESIAN_POINT('Origin',(0.000191696435754032,-0.00799999999999,
-0.0131986079749641));
#31160=CARTESIAN_POINT('',(0.000195327050057368,-0.024,-0.0134485816108434));
#31161=CARTESIAN_POINT('',(0.000195327050067368,-0.00799999999999,-0.0134485816108534));
#31162=CARTESIAN_POINT('',(0.000441556473125542,-0.024,-0.0131902436626865));
#31163=CARTESIAN_POINT('Origin',(0.000191696435754032,-0.02400000000001,
-0.0131986079749641));
#31164=CARTESIAN_POINT('',(0.000441556473135542,-0.00799999999999,-0.0131902436626965));
#31165=CARTESIAN_POINT('Origin',(-4.44089209850063E-17,-0.008,6.72997231505748E-33));
#31166=CARTESIAN_POINT('',(-0.00019532705005746,-0.008,-0.0134485816108434));
#31167=CARTESIAN_POINT('Origin',(-4.44089209850063E-17,-0.00799999999999,
6.72997231505748E-33));
#31168=CARTESIAN_POINT('',(-0.00019532705005746,-0.024,-0.0134485816108434));
#31169=CARTESIAN_POINT('',(-0.00019532705006746,-0.00799999999999,-0.0134485816108534));
#31170=CARTESIAN_POINT('Origin',(-4.44089209850063E-17,-0.02400000000001,
6.72997231505748E-33));
#31171=CARTESIAN_POINT('Origin',(-0.000191696435744125,-0.008,-0.0131986079749541));
#31172=CARTESIAN_POINT('',(-0.000441556473125634,-0.008,-0.0131902436626865));
#31173=CARTESIAN_POINT('Origin',(-0.000191696435754125,-0.00799999999999,
-0.0131986079749641));
#31174=CARTESIAN_POINT('',(-0.000441556473125634,-0.024,-0.0131902436626865));
#31175=CARTESIAN_POINT('',(-0.000441556473135633,-0.00799999999999,-0.0131902436626965));
#31176=CARTESIAN_POINT('Origin',(-0.000191696435754125,-0.02400000000001,
-0.0131986079749641));
#31177=CARTESIAN_POINT('Origin',(-0.000434944237918262,-0.008,-0.0129927219438385));
#31178=CARTESIAN_POINT('',(-0.000434944237918262,-0.008,-0.0129927219438385));
#31179=CARTESIAN_POINT('',(-0.000436112706129081,-0.00799999999999,-0.0130276266077339));
#31180=CARTESIAN_POINT('',(-0.000434944237918262,-0.024,-0.0129927219438385));
#31181=CARTESIAN_POINT('',(-0.000434944237928261,-0.016,-0.0129927219438485));
#31182=CARTESIAN_POINT('',(-0.000436112706129081,-0.02400000000001,-0.0130276266077339));
#31183=CARTESIAN_POINT('Origin',(-0.00153270759541388,-0.008,-0.0131107134598755));
#31184=CARTESIAN_POINT('',(-0.00128389338345847,-0.008,-0.0131350339847262));
#31185=CARTESIAN_POINT('',(-0.00156173614835732,-0.008,-0.0133590224269186));
#31186=CARTESIAN_POINT('Origin',(-0.00153270759542387,-0.00799999999999,
-0.0131107134598855));
#31187=CARTESIAN_POINT('',(-0.00156173614835732,-0.024,-0.0133590224269186));
#31188=CARTESIAN_POINT('',(-0.00156173614836731,-0.00799999999999,-0.0133590224269286));
#31189=CARTESIAN_POINT('',(-0.00128389338345847,-0.024,-0.0131350339847262));
#31190=CARTESIAN_POINT('Origin',(-0.00153270759542387,-0.02400000000001,
-0.0131107134598855));
#31191=CARTESIAN_POINT('',(-0.00128389338346847,-0.00799999999999,-0.0131350339847362));
#31192=CARTESIAN_POINT('Origin',(-4.44089209850063E-17,-0.008,6.72997231505748E-33));
#31193=CARTESIAN_POINT('',(-0.00194904814849077,-0.008,-0.0133080318347555));
#31194=CARTESIAN_POINT('Origin',(-4.44089209850063E-17,-0.00799999999999,
6.72997231505748E-33));
#31195=CARTESIAN_POINT('',(-0.00194904814849077,-0.024,-0.0133080318347555));
#31196=CARTESIAN_POINT('',(-0.00194904814850077,-0.00799999999999,-0.0133080318347655));
#31197=CARTESIAN_POINT('Origin',(-4.44089209850063E-17,-0.02400000000001,
6.72997231505748E-33));
#31198=CARTESIAN_POINT('Origin',(-0.00191282048773815,-0.008,-0.0130606706482359));
#31199=CARTESIAN_POINT('',(-0.00215945117603188,-0.008,-0.0130197646145518));
#31200=CARTESIAN_POINT('Origin',(-0.00191282048774815,-0.00799999999999,
-0.0130606706482459));
#31201=CARTESIAN_POINT('',(-0.00215945117603188,-0.024,-0.0130197646145518));
#31202=CARTESIAN_POINT('',(-0.00215945117604188,-0.00799999999999,-0.0130197646145618));
#31203=CARTESIAN_POINT('Origin',(-0.00191282048774815,-0.02400000000001,
-0.0130606706482459));
#31204=CARTESIAN_POINT('Origin',(-0.00212711375157135,-0.008,-0.0128247957912739));
#31205=CARTESIAN_POINT('',(-0.00212711375157135,-0.008,-0.0128247957912739));
#31206=CARTESIAN_POINT('',(-0.00211900825769018,-0.00799999999999,-0.0127759261415696));
#31207=CARTESIAN_POINT('',(-0.00212711375157135,-0.024,-0.0128247957912739));
#31208=CARTESIAN_POINT('',(-0.00212711375158135,-0.016,-0.0128247957912839));
#31209=CARTESIAN_POINT('',(-0.00211900825769018,-0.02400000000001,-0.0127759261415696));
#31210=CARTESIAN_POINT('Origin',(-0.00323088657466742,-0.008,-0.0127984910025219));
#31211=CARTESIAN_POINT('',(-0.00298737546828901,-0.008,-0.0128550802335678));
#31212=CARTESIAN_POINT('',(-0.00329207760827854,-0.008,-0.0130408866654485));
#31213=CARTESIAN_POINT('Origin',(-0.00323088657467743,-0.00799999999999,
-0.0127984910025319));
#31214=CARTESIAN_POINT('',(-0.00329207760827854,-0.024,-0.0130408866654485));
#31215=CARTESIAN_POINT('',(-0.00329207760828854,-0.00799999999999,-0.0130408866654585));
#31216=CARTESIAN_POINT('',(-0.00298737546828901,-0.024,-0.0128550802335678));
#31217=CARTESIAN_POINT('Origin',(-0.00323088657467743,-0.02400000000001,
-0.0127984910025319));
#31218=CARTESIAN_POINT('',(-0.00298737546829902,-0.00799999999999,-0.0128550802335778));
#31219=CARTESIAN_POINT('Origin',(-4.44089209850063E-17,-0.008,6.72997231505748E-33));
#31220=CARTESIAN_POINT('',(-0.00366942049272517,-0.008,-0.0129397779442914));
#31221=CARTESIAN_POINT('Origin',(-4.44089209850063E-17,-0.00799999999999,
6.72997231505748E-33));
#31222=CARTESIAN_POINT('',(-0.00366942049272517,-0.024,-0.0129397779442914));
#31223=CARTESIAN_POINT('',(-0.00366942049273517,-0.00799999999999,-0.0129397779443014));
#31224=CARTESIAN_POINT('Origin',(-4.44089209850063E-17,-0.02400000000001,
6.72997231505748E-33));
#31225=CARTESIAN_POINT('Origin',(-0.00360121565085296,-0.008,-0.0126992616256242));
#31226=CARTESIAN_POINT('',(-0.00384039707060325,-0.008,-0.0126265137841014));
#31227=CARTESIAN_POINT('Origin',(-0.00360121565086297,-0.00799999999999,
-0.0126992616256342));
#31228=CARTESIAN_POINT('',(-0.00384039707060325,-0.024,-0.0126265137841014));
#31229=CARTESIAN_POINT('',(-0.00384039707061325,-0.00799999999999,-0.0126265137841114));
#31230=CARTESIAN_POINT('Origin',(-0.00360121565086297,-0.02400000000001,
-0.0126992616256342));
#31231=CARTESIAN_POINT('Origin',(-0.0037828877591877,-0.008,-0.0124374338270155));
#31232=CARTESIAN_POINT('',(-0.0037828877591877,-0.008,-0.0124374338270155));
#31233=CARTESIAN_POINT('',(-0.00371177878877267,-0.00799999999999,-0.0122036407116943));
#31234=CARTESIAN_POINT('',(-0.0037828877591877,-0.024,-0.0124374338270155));
#31235=CARTESIAN_POINT('',(-0.00378288775919771,-0.016,-0.0124374338270255));
#31236=CARTESIAN_POINT('',(-0.00371177878877267,-0.02400000000001,-0.0122036407116943));
#31237=CARTESIAN_POINT('Origin',(-0.00304450063026865,-0.008,-0.0131008975231583));
#31238=CARTESIAN_POINT('',(-0.00294264001438606,-0.024,-0.0126625775316771));
#31239=CARTESIAN_POINT('',(-0.00296388861875547,-0.02400000000001,-0.0127540131469256));
#31240=CARTESIAN_POINT('',(-0.00294264001438606,-0.008,-0.0126625775316771));
#31241=CARTESIAN_POINT('',(-0.00294264001439606,-0.016,-0.0126625775316871));
#31242=CARTESIAN_POINT('',(-0.00296388861875547,-0.00799999999999,-0.0127540131469256));
#31243=CARTESIAN_POINT('Origin',(-0.00130844423696623,-0.008,-0.0133862046032006));
#31244=CARTESIAN_POINT('',(-0.00126466729223502,-0.024,-0.0129383390216809));
#31245=CARTESIAN_POINT('',(-0.00128729232076206,-0.02400000000001,-0.0131698072435117));
#31246=CARTESIAN_POINT('',(-0.00126466729223502,-0.008,-0.0129383390216809));
#31247=CARTESIAN_POINT('',(-0.00126466729224502,-0.016,-0.0129383390216909));
#31248=CARTESIAN_POINT('',(-0.00128729232076206,-0.00799999999999,-0.0131698072435117));
#31249=CARTESIAN_POINT('Origin',(0.00220074461220257,-0.008,-0.0132687310302026));
#31250=CARTESIAN_POINT('',(0.00212711375157125,-0.024,-0.0128247957912739));
#31251=CARTESIAN_POINT('',(0.00215582368800574,-0.02400000000001,-0.0129978937610339));
#31252=CARTESIAN_POINT('',(0.00212711375157125,-0.008,-0.0128247957912739));
#31253=CARTESIAN_POINT('',(0.00212711375158126,-0.016,-0.0128247957912839));
#31254=CARTESIAN_POINT('',(0.00215582368800574,-0.00799999999999,-0.0129978937610339));
#31255=CARTESIAN_POINT('Origin',(0.00391383387392873,-0.008,-0.012867960382566));
#31256=CARTESIAN_POINT('',(0.00378288775918762,-0.024,-0.0124374338270155));
#31257=CARTESIAN_POINT('',(0.00377725184614313,-0.02400000000001,-0.0124189039894696));
#31258=CARTESIAN_POINT('',(0.00378288775918762,-0.008,-0.0124374338270155));
#31259=CARTESIAN_POINT('',(0.00378288775919761,-0.016,-0.0124374338270255));
#31260=CARTESIAN_POINT('',(0.00377725184614313,-0.00799999999999,-0.0124189039894696));
#31261=CARTESIAN_POINT('Origin',(-4.44089209850063E-17,-0.016,6.72997231505748E-33));
#31262=CARTESIAN_POINT('',(-0.00433948917003907,-0.008,-0.0122543393841983));
#31263=CARTESIAN_POINT('Origin',(-4.44089209850063E-17,-0.00799999999999,
6.72997231505748E-33));
#31264=CARTESIAN_POINT('',(-0.00433948917003907,-0.024,-0.0122543393841983));
#31265=CARTESIAN_POINT('',(-0.00433948917004907,-0.016,-0.0122543393842083));
#31266=CARTESIAN_POINT('Origin',(-4.44089209850063E-17,-0.02400000000001,
6.72997231505748E-33));
#31267=CARTESIAN_POINT('Origin',(-4.44089209850063E-17,-0.016,6.72997231505748E-33));
#31268=CARTESIAN_POINT('Origin',(-4.44089209850063E-17,-0.02400000000001,
6.72997231505748E-33));
#31269=CARTESIAN_POINT('Origin',(-4.44089209850063E-17,-0.00799999999999,
6.72997231505748E-33));
#31270=CARTESIAN_POINT('Origin',(-4.57966997657877E-17,-0.024,-0.0130771696920992));
#31271=CARTESIAN_POINT('',(-0.00463991534334946,-0.024,-0.0131027167261813));
#31272=CARTESIAN_POINT('',(-0.00463991534335947,-0.02400000000001,-0.0131027167261913));
#31273=CARTESIAN_POINT('',(0.00463991534334938,-0.024,-0.0131027167261813));
#31274=CARTESIAN_POINT('Origin',(-4.44089209850063E-17,-0.02400000000001,
6.72997231505748E-33));
#31275=CARTESIAN_POINT('',(0.00433948917003898,-0.024,-0.0122543393841983));
#31276=CARTESIAN_POINT('',(0.00433948917004898,-0.02400000000001,-0.0122543393842083));
#31277=CARTESIAN_POINT('Origin',(-4.44089209850063E-17,-0.02400000000001,
6.72997231505748E-33));
#31278=CARTESIAN_POINT('Origin',(-4.44089209850063E-17,-0.02400000000001,
6.72997231505748E-33));
#31279=CARTESIAN_POINT('',(0.00043494423791817,-0.024,-0.0129927219438385));
#31280=CARTESIAN_POINT('Origin',(-4.44089209850063E-17,-0.02400000000001,
6.72997231505748E-33));
#31281=CARTESIAN_POINT('',(0.000443640587169881,-0.02400000000001,-0.0132525006413773));
#31282=CARTESIAN_POINT('Origin',(-4.44089209850063E-17,-0.02400000000001,
6.72997231505748E-33));
#31283=CARTESIAN_POINT('Origin',(-4.44089209850063E-17,-0.016,6.72997231505748E-33));
#31284=CARTESIAN_POINT('',(0.00043494423791817,-0.008,-0.0129927219438385));
#31285=CARTESIAN_POINT('Origin',(-4.44089209850063E-17,-0.00799999999999,
6.72997231505748E-33));
#31286=CARTESIAN_POINT('',(0.00043494423792817,-0.016,-0.0129927219438485));
#31287=CARTESIAN_POINT('Origin',(-4.44089209850063E-17,-0.016,6.72997231505748E-33));
#31288=CARTESIAN_POINT('',(0.00433948917003898,-0.008,-0.0122543393841983));
#31289=CARTESIAN_POINT('',(0.00433948917004898,-0.016,-0.0122543393842083));
#31290=CARTESIAN_POINT('Origin',(-4.44089209850063E-17,-0.00799999999999,
6.72997231505748E-33));
#31291=CARTESIAN_POINT('Origin',(0.000449999999999955,-0.008,-0.0134424700111252));
#31292=CARTESIAN_POINT('',(0.000443640587169881,-0.00799999999999,-0.0132525006413773));
#31293=CARTESIAN_POINT('Origin',(-4.44089209850063E-17,-0.016,6.72997231505748E-33));
#31294=CARTESIAN_POINT('Origin',(-4.44089209850063E-17,-0.00799999999999,
6.72997231505748E-33));
#31295=CARTESIAN_POINT('Origin',(-0.00463991534334946,-0.016,-0.0131027167261813));
#31296=CARTESIAN_POINT('',(-0.00463991534334946,-0.008,-0.0131027167261813));
#31297=CARTESIAN_POINT('',(-0.00463991534335947,-0.00799999999999,-0.0131027167261913));
#31298=CARTESIAN_POINT('',(-0.00463991534335947,-0.016,-0.0131027167261913));
#31299=CARTESIAN_POINT('Origin',(-4.44089209850063E-17,-0.016,6.72997231505748E-33));
#31300=CARTESIAN_POINT('',(0.00463991534334938,-0.008,-0.0131027167261813));
#31301=CARTESIAN_POINT('Origin',(-4.44089209850063E-17,-0.00799999999999,
6.72997231505748E-33));
#31302=CARTESIAN_POINT('',(0.00463991534335938,-0.016,-0.0131027167261913));
#31303=CARTESIAN_POINT('Origin',(0.00433948917003898,-0.016,-0.0122543393841983));
#31304=CARTESIAN_POINT('',(0.00433948917004898,-0.00799999999999,-0.0122543393842083));
#31305=CARTESIAN_POINT('Origin',(-4.44089209850063E-17,-0.016,6.72997231505748E-33));
#31306=CARTESIAN_POINT('Origin',(-4.44089209850063E-17,-0.00799999999999,
6.72997231505748E-33));
#31307=CARTESIAN_POINT('Origin',(-4.57966997657877E-17,-0.008,-0.0130771696920992));
#34818=UNCERTAINTY_MEASURE_WITH_UNIT(LENGTH_MEASURE(1.E-5),#34877,
'DISTANCE_ACCURACY_VALUE',
'Maximum model space distance between geometric entities at asserted c
onnectivities');
#34841=UNCERTAINTY_MEASURE_WITH_UNIT(LENGTH_MEASURE(1.E-5),#34877,
'DISTANCE_ACCURACY_VALUE',
'Maximum model space distance between geometric entities at asserted c
onnectivities');
#34853=(
GEOMETRIC_REPRESENTATION_CONTEXT(3)
GLOBAL_UNCERTAINTY_ASSIGNED_CONTEXT((#34818))
GLOBAL_UNIT_ASSIGNED_CONTEXT((#34877,#34878,#34879))
REPRESENTATION_CONTEXT('','3D')
);
#34876=(
GEOMETRIC_REPRESENTATION_CONTEXT(3)
GLOBAL_UNCERTAINTY_ASSIGNED_CONTEXT((#34841))
GLOBAL_UNIT_ASSIGNED_CONTEXT((#34877,#34878,#34879))
REPRESENTATION_CONTEXT('','3D')
);
#34877=(
LENGTH_UNIT()
NAMED_UNIT(*)
SI_UNIT($,.METRE.)
);
#34878=(
NAMED_UNIT(*)
PLANE_ANGLE_UNIT()
SI_UNIT($,.RADIAN.)
);
#34879=(
NAMED_UNIT(*)
SI_UNIT($,.STERADIAN.)
SOLID_ANGLE_UNIT()
);
#34891=SHAPE_DEFINITION_REPRESENTATION(#34925,#34995);
#34925=PRODUCT_DEFINITION_SHAPE('',$,#35030);
#34995=SHAPE_REPRESENTATION('',(#20884),#34853);
#35018=PRODUCT_DEFINITION_CONTEXT('part definition',#35122,'design');
#35030=PRODUCT_DEFINITION('Motor Stator Face 2','Motor Stator Face 2',#35064,
#35018);
#35064=PRODUCT_DEFINITION_FORMATION('',$,#35135);
#35122=APPLICATION_CONTEXT('Managed model based 3d engineering');
#35123=PRODUCT_CONTEXT('part definition',#35122,'mechanical');
#35135=PRODUCT('Motor Stator Face 2','Motor Stator Face 2',
'LEGAL AND USAGE DISCLAIMER: this Data/Model is provided \X2\201C\X0\A
S IS\X2\201D\X0\ for informational and representational only. It is a 
geometric approximation and is NOT engineered, certified, or guarantee
d for dimensional accuracy, exact tolerances, or production-level prec
ision. Vendor disclaims all implied warranties including fitness for a
 particular purpose. DO NOT USE FOR DIRECT PHYSICAL MANUFACTURING, AUT
OMATED PRODUCTION, OR SAFETY-CRITICAL SYSTEMS without independent engi
neering verification and resolution of any design discrepancies.',(#35123));
#35166=PRESENTATION_STYLE_ASSIGNMENT((#35175));
#35175=SURFACE_STYLE_USAGE(.BOTH.,#35184);
#35184=SURFACE_SIDE_STYLE('',(#35193));
#35193=SURFACE_STYLE_FILL_AREA(#35202);
#35202=FILL_AREA_STYLE('Paint - Enamel Glossy (Grey)',(#35211));
#35211=FILL_AREA_STYLE_COLOUR('Paint - Enamel Glossy (Grey)',#35220);
#35220=COLOUR_RGB('Paint - Enamel Glossy (Grey)',0.701960784313725,0.701960784313725,
0.701960784313725);
ENDSEC;
END-ISO-10303-21;
